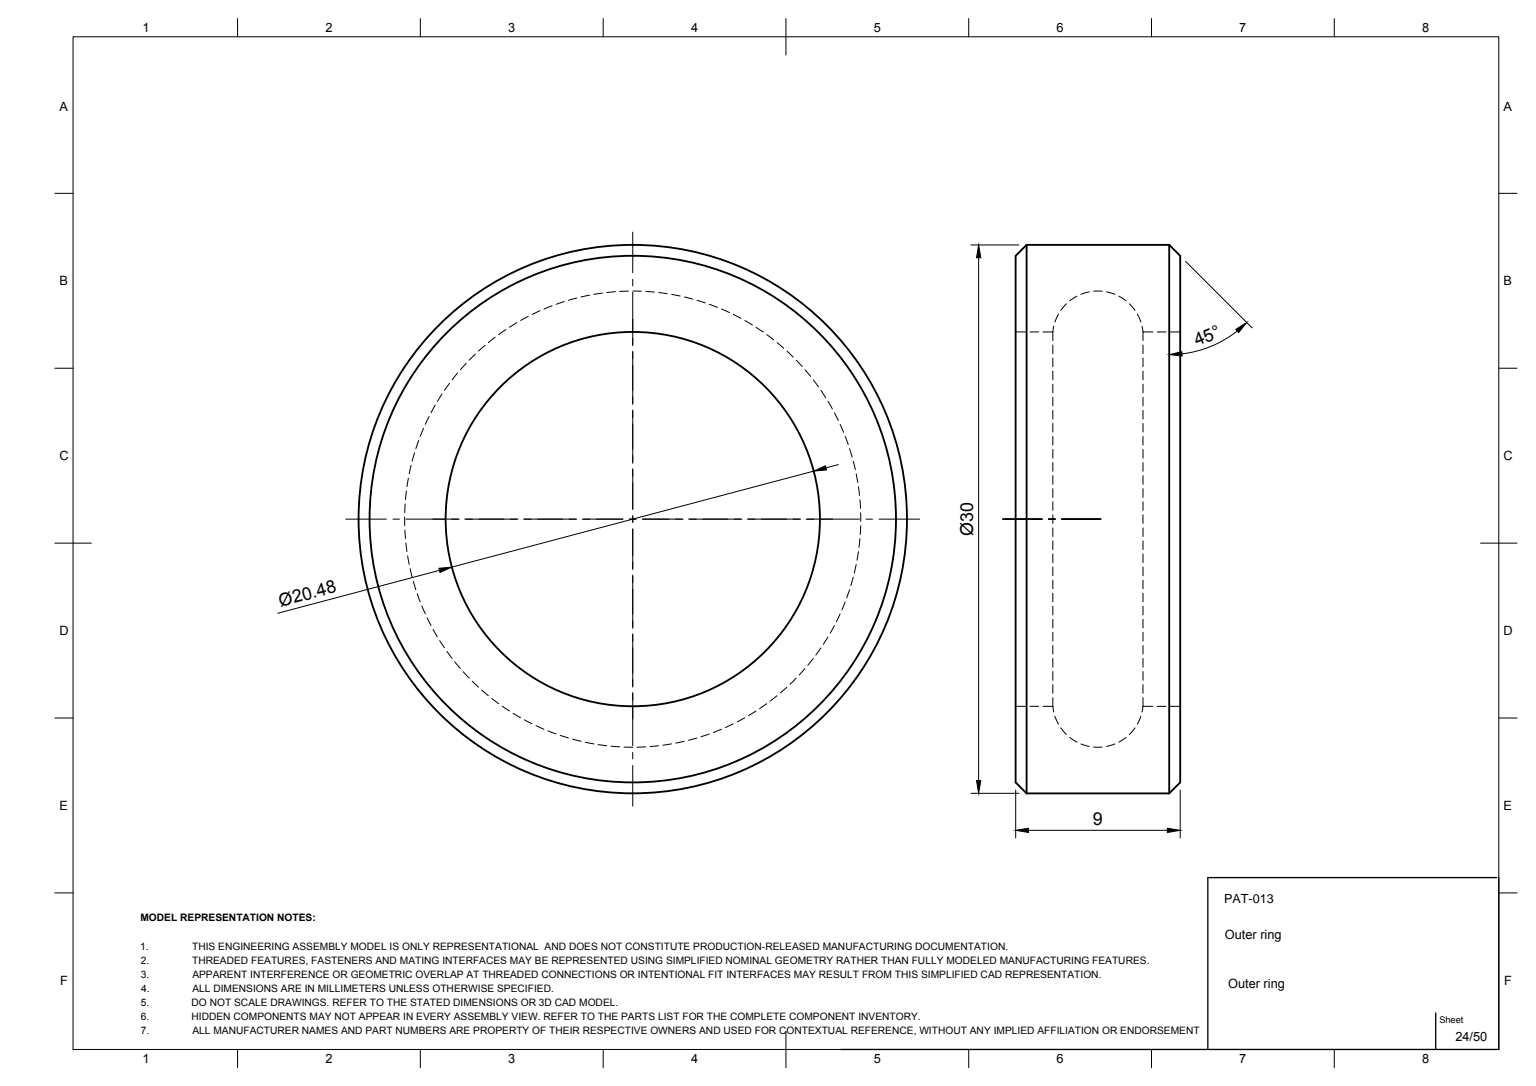
ISO-10303-21;
HEADER;
/* Generated by software containing ST-Developer
 * from STEP Tools, Inc. (www.steptools.com) 
 */

FILE_DESCRIPTION(
/* description */ ('Belt-driven linear axis on 2020 extrusion'),
/* implementation_level */ '2;1');

FILE_NAME(
/* name */ 'Outer ring.step',
/* time_stamp */ '2026-10-28T03:26:09-07:00',
/* author */ (''),
/* organization */ (''),
/* preprocessor_version */ 'ST-DEVELOPER v20.2',
/* originating_system */ 'Autodesk Translation Framework v15.17.0.0',
/* authorisation */ '');

FILE_SCHEMA (('AUTOMOTIVE_DESIGN { 1 0 10303 214 3 1 1 }'));
ENDSEC;

DATA;
#10=MECHANICAL_DESIGN_GEOMETRIC_PRESENTATION_REPRESENTATION('',(#627),#20096);
#499=CONICAL_SURFACE('',#11949,1.47,0.785398163397449);
#500=CONICAL_SURFACE('',#11953,1.47,0.785398163397449);
#517=TOROIDAL_SURFACE('',#11938,1.,0.247676);
#533=SHAPE_REPRESENTATION_RELATIONSHIP('SRR','None',#20330,#579);
#579=ADVANCED_BREP_SHAPE_REPRESENTATION('',(#683),#20061);
#627=STYLED_ITEM('',(#20650),#683);
#683=MANIFOLD_SOLID_BREP('Body1',#10940);
#806=FACE_BOUND('',#2185,.T.);
#807=FACE_BOUND('',#2190,.T.);
#1007=PLANE('',#11946);
#1008=PLANE('',#11955);
#1472=FACE_OUTER_BOUND('',#2182,.T.);
#1473=FACE_OUTER_BOUND('',#2183,.T.);
#1474=FACE_OUTER_BOUND('',#2184,.T.);
#1475=FACE_OUTER_BOUND('',#2186,.T.);
#1476=FACE_OUTER_BOUND('',#2187,.T.);
#1477=FACE_OUTER_BOUND('',#2188,.T.);
#1478=FACE_OUTER_BOUND('',#2189,.T.);
#1479=FACE_OUTER_BOUND('',#2191,.T.);
#2182=EDGE_LOOP('',(#8257,#8258,#8259,#8260,#8261,#8262));
#2183=EDGE_LOOP('',(#8263,#8264,#8265,#8266,#8267));
#2184=EDGE_LOOP('',(#8268));
#2185=EDGE_LOOP('',(#8269));
#2186=EDGE_LOOP('',(#8270,#8271,#8272,#8273));
#2187=EDGE_LOOP('',(#8274,#8275,#8276,#8277));
#2188=EDGE_LOOP('',(#8278,#8279,#8280,#8281));
#2189=EDGE_LOOP('',(#8282));
#2190=EDGE_LOOP('',(#8283));
#2191=EDGE_LOOP('',(#8284,#8285,#8286,#8287,#8288));
#2960=LINE('',#17322,#3817);
#2961=LINE('',#17331,#3818);
#2962=LINE('',#17335,#3819);
#2963=LINE('',#17339,#3820);
#2964=LINE('',#17342,#3821);
#3817=VECTOR('',#13992,1.023815);
#3818=VECTOR('',#14003,1.47);
#3819=VECTOR('',#14008,1.5);
#3820=VECTOR('',#14013,1.47);
#3821=VECTOR('',#14018,1.023815);
#4586=CIRCLE('',#11939,1.023815);
#4587=CIRCLE('',#11940,1.023815);
#4588=CIRCLE('',#11941,0.247676);
#4589=CIRCLE('',#11942,1.023815);
#4590=CIRCLE('',#11943,1.023815);
#4591=CIRCLE('',#11945,1.023815);
#4592=CIRCLE('',#11947,1.44);
#4593=CIRCLE('',#11948,1.023815);
#4594=CIRCLE('',#11950,1.5);
#4595=CIRCLE('',#11952,1.5);
#4596=CIRCLE('',#11954,1.44);
#5226=VERTEX_POINT('',#17310);
#5227=VERTEX_POINT('',#17311);
#5228=VERTEX_POINT('',#17314);
#5229=VERTEX_POINT('',#17316);
#5230=VERTEX_POINT('',#17320);
#5231=VERTEX_POINT('',#17324);
#5232=VERTEX_POINT('',#17326);
#5233=VERTEX_POINT('',#17329);
#5234=VERTEX_POINT('',#17333);
#5235=VERTEX_POINT('',#17337);
#6343=EDGE_CURVE('',#5226,#5227,#4586,.T.);
#6344=EDGE_CURVE('',#5227,#5226,#4587,.T.);
#6345=EDGE_CURVE('',#5227,#5228,#4588,.T.);
#6346=EDGE_CURVE('',#5229,#5228,#4589,.T.);
#6347=EDGE_CURVE('',#5228,#5229,#4590,.T.);
#6348=EDGE_CURVE('',#5230,#5230,#4591,.T.);
#6349=EDGE_CURVE('',#5230,#5229,#2960,.T.);
#6350=EDGE_CURVE('',#5231,#5231,#4592,.T.);
#6351=EDGE_CURVE('',#5232,#5232,#4593,.T.);
#6352=EDGE_CURVE('',#5233,#5233,#4594,.T.);
#6353=EDGE_CURVE('',#5233,#5231,#2961,.T.);
#6354=EDGE_CURVE('',#5234,#5234,#4595,.T.);
#6355=EDGE_CURVE('',#5234,#5233,#2962,.T.);
#6356=EDGE_CURVE('',#5235,#5235,#4596,.T.);
#6357=EDGE_CURVE('',#5235,#5234,#2963,.T.);
#6358=EDGE_CURVE('',#5226,#5232,#2964,.T.);
#8257=ORIENTED_EDGE('',*,*,#6343,.F.);
#8258=ORIENTED_EDGE('',*,*,#6344,.F.);
#8259=ORIENTED_EDGE('',*,*,#6345,.T.);
#8260=ORIENTED_EDGE('',*,*,#6346,.F.);
#8261=ORIENTED_EDGE('',*,*,#6347,.F.);
#8262=ORIENTED_EDGE('',*,*,#6345,.F.);
#8263=ORIENTED_EDGE('',*,*,#6348,.T.);
#8264=ORIENTED_EDGE('',*,*,#6349,.T.);
#8265=ORIENTED_EDGE('',*,*,#6346,.T.);
#8266=ORIENTED_EDGE('',*,*,#6347,.T.);
#8267=ORIENTED_EDGE('',*,*,#6349,.F.);
#8268=ORIENTED_EDGE('',*,*,#6350,.F.);
#8269=ORIENTED_EDGE('',*,*,#6351,.T.);
#8270=ORIENTED_EDGE('',*,*,#6352,.F.);
#8271=ORIENTED_EDGE('',*,*,#6353,.T.);
#8272=ORIENTED_EDGE('',*,*,#6350,.T.);
#8273=ORIENTED_EDGE('',*,*,#6353,.F.);
#8274=ORIENTED_EDGE('',*,*,#6354,.F.);
#8275=ORIENTED_EDGE('',*,*,#6355,.T.);
#8276=ORIENTED_EDGE('',*,*,#6352,.T.);
#8277=ORIENTED_EDGE('',*,*,#6355,.F.);
#8278=ORIENTED_EDGE('',*,*,#6356,.F.);
#8279=ORIENTED_EDGE('',*,*,#6357,.T.);
#8280=ORIENTED_EDGE('',*,*,#6354,.T.);
#8281=ORIENTED_EDGE('',*,*,#6357,.F.);
#8282=ORIENTED_EDGE('',*,*,#6356,.T.);
#8283=ORIENTED_EDGE('',*,*,#6348,.F.);
#8284=ORIENTED_EDGE('',*,*,#6343,.T.);
#8285=ORIENTED_EDGE('',*,*,#6344,.T.);
#8286=ORIENTED_EDGE('',*,*,#6358,.T.);
#8287=ORIENTED_EDGE('',*,*,#6351,.F.);
#8288=ORIENTED_EDGE('',*,*,#6358,.F.);
#10178=CYLINDRICAL_SURFACE('',#11944,1.023815);
#10179=CYLINDRICAL_SURFACE('',#11951,1.5);
#10180=CYLINDRICAL_SURFACE('',#11956,1.023815);
#10523=ADVANCED_FACE('',(#1472),#517,.F.);
#10524=ADVANCED_FACE('',(#1473),#10178,.F.);
#10525=ADVANCED_FACE('',(#1474,#806),#1007,.T.);
#10526=ADVANCED_FACE('',(#1475),#499,.T.);
#10527=ADVANCED_FACE('',(#1476),#10179,.T.);
#10528=ADVANCED_FACE('',(#1477),#500,.T.);
#10529=ADVANCED_FACE('',(#1478,#807),#1008,.T.);
#10530=ADVANCED_FACE('',(#1479),#10180,.F.);
#10940=CLOSED_SHELL('',(#10523,#10524,#10525,#10526,#10527,#10528,#10529,
#10530));
#11937=AXIS2_PLACEMENT_3D('',#17308,#13974,#13975);
#11938=AXIS2_PLACEMENT_3D('',#17309,#13976,#13977);
#11939=AXIS2_PLACEMENT_3D('',#17312,#13978,#13979);
#11940=AXIS2_PLACEMENT_3D('',#17313,#13980,#13981);
#11941=AXIS2_PLACEMENT_3D('',#17315,#13982,#13983);
#11942=AXIS2_PLACEMENT_3D('',#17317,#13984,#13985);
#11943=AXIS2_PLACEMENT_3D('',#17318,#13986,#13987);
#11944=AXIS2_PLACEMENT_3D('',#17319,#13988,#13989);
#11945=AXIS2_PLACEMENT_3D('',#17321,#13990,#13991);
#11946=AXIS2_PLACEMENT_3D('',#17323,#13993,#13994);
#11947=AXIS2_PLACEMENT_3D('',#17325,#13995,#13996);
#11948=AXIS2_PLACEMENT_3D('',#17327,#13997,#13998);
#11949=AXIS2_PLACEMENT_3D('',#17328,#13999,#14000);
#11950=AXIS2_PLACEMENT_3D('',#17330,#14001,#14002);
#11951=AXIS2_PLACEMENT_3D('',#17332,#14004,#14005);
#11952=AXIS2_PLACEMENT_3D('',#17334,#14006,#14007);
#11953=AXIS2_PLACEMENT_3D('',#17336,#14009,#14010);
#11954=AXIS2_PLACEMENT_3D('',#17338,#14011,#14012);
#11955=AXIS2_PLACEMENT_3D('',#17340,#14014,#14015);
#11956=AXIS2_PLACEMENT_3D('',#17341,#14016,#14017);
#13974=DIRECTION('axis',(0.,0.,1.));
#13975=DIRECTION('refdir',(1.,0.,0.));
#13976=DIRECTION('center_axis',(0.,-1.,0.));
#13977=DIRECTION('ref_axis',(0.,0.,-1.));
#13978=DIRECTION('center_axis',(0.,-1.,0.));
#13979=DIRECTION('ref_axis',(1.,0.,0.));
#13980=DIRECTION('center_axis',(0.,-1.,0.));
#13981=DIRECTION('ref_axis',(1.,0.,0.));
#13982=DIRECTION('center_axis',(1.,0.,1.22464679914735E-16));
#13983=DIRECTION('ref_axis',(-1.22464679914735E-16,0.,1.));
#13984=DIRECTION('center_axis',(0.,1.,0.));
#13985=DIRECTION('ref_axis',(1.,0.,0.));
#13986=DIRECTION('center_axis',(0.,1.,0.));
#13987=DIRECTION('ref_axis',(1.,0.,0.));
#13988=DIRECTION('center_axis',(0.,-1.,0.));
#13989=DIRECTION('ref_axis',(1.,0.,0.));
#13990=DIRECTION('center_axis',(0.,-1.,0.));
#13991=DIRECTION('ref_axis',(1.,0.,0.));
#13992=DIRECTION('',(0.,1.,0.));
#13993=DIRECTION('center_axis',(0.,1.,0.));
#13994=DIRECTION('ref_axis',(0.,0.,1.));
#13995=DIRECTION('center_axis',(0.,-1.,0.));
#13996=DIRECTION('ref_axis',(1.,0.,0.));
#13997=DIRECTION('center_axis',(0.,-1.,0.));
#13998=DIRECTION('ref_axis',(1.,0.,0.));
#13999=DIRECTION('center_axis',(0.,-1.,0.));
#14000=DIRECTION('ref_axis',(1.,0.,0.));
#14001=DIRECTION('center_axis',(0.,-1.,0.));
#14002=DIRECTION('ref_axis',(1.,0.,0.));
#14003=DIRECTION('',(0.707106781186548,0.707106781186547,8.65956056235494E-17));
#14004=DIRECTION('center_axis',(0.,-1.,0.));
#14005=DIRECTION('ref_axis',(1.,0.,0.));
#14006=DIRECTION('center_axis',(0.,-1.,0.));
#14007=DIRECTION('ref_axis',(1.,0.,0.));
#14008=DIRECTION('',(0.,1.,0.));
#14009=DIRECTION('center_axis',(0.,1.,0.));
#14010=DIRECTION('ref_axis',(1.,0.,0.));
#14011=DIRECTION('center_axis',(0.,-1.,0.));
#14012=DIRECTION('ref_axis',(1.,0.,0.));
#14013=DIRECTION('',(-0.707106781186548,0.707106781186547,-8.65956056235494E-17));
#14014=DIRECTION('center_axis',(0.,-1.,0.));
#14015=DIRECTION('ref_axis',(0.,0.,-1.));
#14016=DIRECTION('center_axis',(0.,-1.,0.));
#14017=DIRECTION('ref_axis',(1.,0.,0.));
#14018=DIRECTION('',(0.,1.,0.));
#17308=CARTESIAN_POINT('',(0.,0.,0.));
#17309=CARTESIAN_POINT('Origin',(0.,0.,0.));
#17310=CARTESIAN_POINT('',(-1.023815,0.246528389340863,-1.25381176266905E-16));
#17311=CARTESIAN_POINT('',(-1.25381176266905E-16,0.246528389340863,1.023815));
#17312=CARTESIAN_POINT('Origin',(0.,0.246528389340863,0.));
#17313=CARTESIAN_POINT('Origin',(0.,0.246528389340863,0.));
#17314=CARTESIAN_POINT('',(-1.25381176266905E-16,-0.246528389340863,1.023815));
#17315=CARTESIAN_POINT('Origin',(-1.22464679914735E-16,0.,1.));
#17316=CARTESIAN_POINT('',(-1.023815,-0.246528389340863,1.25381176266905E-16));
#17317=CARTESIAN_POINT('Origin',(0.,-0.246528389340863,0.));
#17318=CARTESIAN_POINT('Origin',(0.,-0.246528389340863,0.));
#17319=CARTESIAN_POINT('Origin',(0.,0.,0.));
#17320=CARTESIAN_POINT('',(-1.023815,-0.45,-1.25381176266905E-16));
#17321=CARTESIAN_POINT('Origin',(0.,-0.45,0.));
#17322=CARTESIAN_POINT('',(-1.023815,0.,-1.25381176266905E-16));
#17323=CARTESIAN_POINT('Origin',(1.44,0.45,0.));
#17324=CARTESIAN_POINT('',(-1.44,0.45,-1.76349139077219E-16));
#17325=CARTESIAN_POINT('Origin',(0.,0.45,0.));
#17326=CARTESIAN_POINT('',(-1.023815,0.45,-1.25381176266905E-16));
#17327=CARTESIAN_POINT('Origin',(0.,0.45,0.));
#17328=CARTESIAN_POINT('Origin',(0.,0.42,0.));
#17329=CARTESIAN_POINT('',(-1.5,0.39,-1.83697019872103E-16));
#17330=CARTESIAN_POINT('Origin',(0.,0.39,0.));
#17331=CARTESIAN_POINT('',(-1.47,0.42,-1.80023079474661E-16));
#17332=CARTESIAN_POINT('Origin',(0.,0.,0.));
#17333=CARTESIAN_POINT('',(-1.5,-0.39,-1.83697019872103E-16));
#17334=CARTESIAN_POINT('Origin',(0.,-0.39,0.));
#17335=CARTESIAN_POINT('',(-1.5,0.,-1.83697019872103E-16));
#17336=CARTESIAN_POINT('Origin',(0.,-0.42,0.));
#17337=CARTESIAN_POINT('',(-1.44,-0.45,-1.76349139077219E-16));
#17338=CARTESIAN_POINT('Origin',(0.,-0.45,0.));
#17339=CARTESIAN_POINT('',(-1.47,-0.42,-1.80023079474661E-16));
#17340=CARTESIAN_POINT('Origin',(1.023815,-0.45,0.));
#17341=CARTESIAN_POINT('Origin',(0.,0.,0.));
#17342=CARTESIAN_POINT('',(-1.023815,0.,-1.25381176266905E-16));
#20007=UNCERTAINTY_MEASURE_WITH_UNIT(LENGTH_MEASURE(0.001),#20097,
'DISTANCE_ACCURACY_VALUE',
'Maximum model space distance between geometric entities at asserted c
onnectivities');
#20042=UNCERTAINTY_MEASURE_WITH_UNIT(LENGTH_MEASURE(0.001),#20097,
'DISTANCE_ACCURACY_VALUE',
'Maximum model space distance between geometric entities at asserted c
onnectivities');
#20061=(
GEOMETRIC_REPRESENTATION_CONTEXT(3)
GLOBAL_UNCERTAINTY_ASSIGNED_CONTEXT((#20007))
GLOBAL_UNIT_ASSIGNED_CONTEXT((#20097,#20099,#20100))
REPRESENTATION_CONTEXT('','3D')
);
#20096=(
GEOMETRIC_REPRESENTATION_CONTEXT(3)
GLOBAL_UNCERTAINTY_ASSIGNED_CONTEXT((#20042))
GLOBAL_UNIT_ASSIGNED_CONTEXT((#20097,#20099,#20100))
REPRESENTATION_CONTEXT('','3D')
);
#20097=(
LENGTH_UNIT()
NAMED_UNIT(*)
SI_UNIT(.CENTI.,.METRE.)
);
#20099=(
NAMED_UNIT(*)
PLANE_ANGLE_UNIT()
SI_UNIT($,.RADIAN.)
);
#20100=(
NAMED_UNIT(*)
SI_UNIT($,.STERADIAN.)
SOLID_ANGLE_UNIT()
);
#20119=SHAPE_DEFINITION_REPRESENTATION(#20172,#20330);
#20172=PRODUCT_DEFINITION_SHAPE('',$,#20384);
#20330=SHAPE_REPRESENTATION('',(#11937),#20061);
#20365=PRODUCT_DEFINITION_CONTEXT('part definition',#20526,'design');
#20384=PRODUCT_DEFINITION('Outer ring','Outer ring',#20437,#20365);
#20437=PRODUCT_DEFINITION_FORMATION('',$,#20546);
#20526=APPLICATION_CONTEXT(
'Core Data for Automotive Mechanical Design Process');
#20527=PRODUCT_CONTEXT('part definition',#20526,'mechanical');
#20546=PRODUCT('Outer ring','Outer ring','Outer ring',(#20527));
#20644=COLOUR_RGB('Grey',0.48,0.52,0.57);
#20645=FILL_AREA_STYLE_COLOUR('',#20644);
#20646=FILL_AREA_STYLE('',(#20645));
#20647=SURFACE_STYLE_FILL_AREA(#20646);
#20648=SURFACE_SIDE_STYLE('',(#20647));
#20649=SURFACE_STYLE_USAGE(.BOTH.,#20648);
#20650=PRESENTATION_STYLE_ASSIGNMENT((#20649));
ENDSEC;
END-ISO-10303-21;
